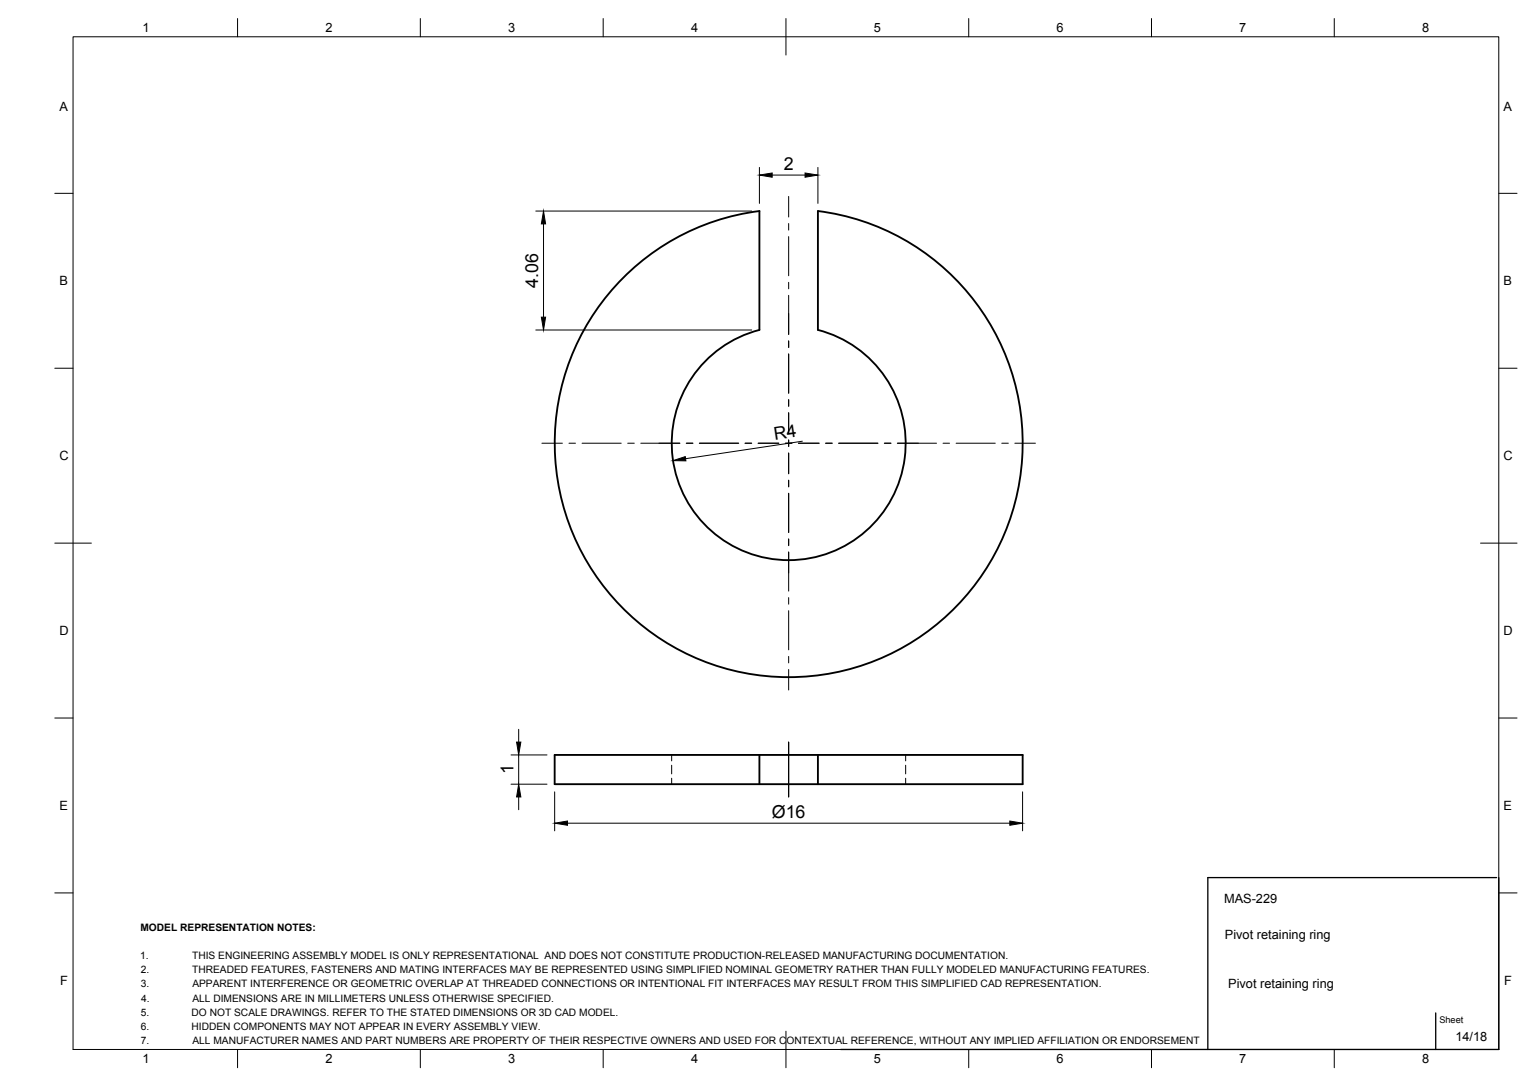
ISO-10303-21;
HEADER;
/* Generated by software containing ST-Developer
 * from STEP Tools, Inc. (www.steptools.com) 
 */

FILE_DESCRIPTION(
/* description */ ('Independently dimensioned six-bar single-leg walking-linkage demonstr
ator. Whole-mm20 crank,60 upper rocker,80/120 ternary coupler,120 lowe
r rocker,140 knee pitch and260 toe reach; ground pivots0/0,60/0,40/60.
 Seven native revolutes close both loops. Four reused native library f
amilies, fully retained shared pins and layered real spacer stacks, bo
nded rubber toe. Benchtop reference mechanism; no complete vehicle, lo
ad, gait stability, adhesive, weld, fit or life rating.'),
/* implementation_level */ '2;1');

FILE_NAME(
/* name */ 'Pivot retaining ring.step',
/* time_stamp */ '2026-11-09T20:33:14-08:00',
/* author */ (''),
/* organization */ (''),
/* preprocessor_version */ 'ST-DEVELOPER v20.2',
/* originating_system */ 'Autodesk Translation Framework v15.17.0.0',
/* authorisation */ '');

FILE_SCHEMA (('AUTOMOTIVE_DESIGN { 1 0 10303 214 3 1 1 }'));
ENDSEC;

DATA;
#10=MECHANICAL_DESIGN_GEOMETRIC_PRESENTATION_REPRESENTATION('',(#269),#4048);
#233=SHAPE_REPRESENTATION_RELATIONSHIP('SRR','None',#4157,#251);
#251=ADVANCED_BREP_SHAPE_REPRESENTATION('',(#287),#4044);
#269=STYLED_ITEM('',(#4254),#287);
#287=MANIFOLD_SOLID_BREP('Body1',#2158);
#402=PLANE('',#2574);
#403=PLANE('',#2575);
#404=PLANE('',#2576);
#405=PLANE('',#2583);
#518=FACE_OUTER_BOUND('',#694,.T.);
#519=FACE_OUTER_BOUND('',#695,.T.);
#520=FACE_OUTER_BOUND('',#696,.T.);
#521=FACE_OUTER_BOUND('',#697,.T.);
#522=FACE_OUTER_BOUND('',#698,.T.);
#523=FACE_OUTER_BOUND('',#699,.T.);
#694=EDGE_LOOP('',(#1891,#1892,#1893,#1894));
#695=EDGE_LOOP('',(#1895,#1896,#1897,#1898));
#696=EDGE_LOOP('',(#1899,#1900,#1901,#1902));
#697=EDGE_LOOP('',(#1903,#1904,#1905,#1906));
#698=EDGE_LOOP('',(#1907,#1908,#1909,#1910));
#699=EDGE_LOOP('',(#1911,#1912,#1913,#1914));
#833=LINE('',#3875,#958);
#834=LINE('',#3877,#959);
#835=LINE('',#3879,#960);
#836=LINE('',#3880,#961);
#837=LINE('',#3884,#962);
#838=LINE('',#3886,#963);
#839=LINE('',#3888,#964);
#840=LINE('',#3889,#965);
#958=VECTOR('',#3208,10.);
#959=VECTOR('',#3209,10.);
#960=VECTOR('',#3210,10.);
#961=VECTOR('',#3211,10.);
#962=VECTOR('',#3214,10.);
#963=VECTOR('',#3215,10.);
#964=VECTOR('',#3216,10.);
#965=VECTOR('',#3217,10.);
#1068=CIRCLE('',#2577,8.);
#1069=CIRCLE('',#2578,4.);
#1070=CIRCLE('',#2580,4.);
#1071=CIRCLE('',#2582,8.);
#1222=VERTEX_POINT('',#3873);
#1223=VERTEX_POINT('',#3874);
#1224=VERTEX_POINT('',#3876);
#1225=VERTEX_POINT('',#3878);
#1226=VERTEX_POINT('',#3882);
#1227=VERTEX_POINT('',#3883);
#1228=VERTEX_POINT('',#3885);
#1229=VERTEX_POINT('',#3887);
#1449=EDGE_CURVE('',#1222,#1223,#833,.T.);
#1450=EDGE_CURVE('',#1224,#1222,#834,.T.);
#1451=EDGE_CURVE('',#1225,#1224,#835,.T.);
#1452=EDGE_CURVE('',#1223,#1225,#836,.T.);
#1453=EDGE_CURVE('',#1226,#1227,#837,.T.);
#1454=EDGE_CURVE('',#1228,#1226,#838,.T.);
#1455=EDGE_CURVE('',#1229,#1228,#839,.T.);
#1456=EDGE_CURVE('',#1227,#1229,#840,.T.);
#1457=EDGE_CURVE('',#1224,#1229,#1068,.T.);
#1458=EDGE_CURVE('',#1227,#1222,#1069,.T.);
#1459=EDGE_CURVE('',#1226,#1223,#1070,.T.);
#1460=EDGE_CURVE('',#1225,#1228,#1071,.T.);
#1891=ORIENTED_EDGE('',*,*,#1449,.F.);
#1892=ORIENTED_EDGE('',*,*,#1450,.F.);
#1893=ORIENTED_EDGE('',*,*,#1451,.F.);
#1894=ORIENTED_EDGE('',*,*,#1452,.F.);
#1895=ORIENTED_EDGE('',*,*,#1453,.F.);
#1896=ORIENTED_EDGE('',*,*,#1454,.F.);
#1897=ORIENTED_EDGE('',*,*,#1455,.F.);
#1898=ORIENTED_EDGE('',*,*,#1456,.F.);
#1899=ORIENTED_EDGE('',*,*,#1456,.T.);
#1900=ORIENTED_EDGE('',*,*,#1457,.F.);
#1901=ORIENTED_EDGE('',*,*,#1450,.T.);
#1902=ORIENTED_EDGE('',*,*,#1458,.F.);
#1903=ORIENTED_EDGE('',*,*,#1453,.T.);
#1904=ORIENTED_EDGE('',*,*,#1458,.T.);
#1905=ORIENTED_EDGE('',*,*,#1449,.T.);
#1906=ORIENTED_EDGE('',*,*,#1459,.F.);
#1907=ORIENTED_EDGE('',*,*,#1455,.T.);
#1908=ORIENTED_EDGE('',*,*,#1460,.F.);
#1909=ORIENTED_EDGE('',*,*,#1451,.T.);
#1910=ORIENTED_EDGE('',*,*,#1457,.T.);
#1911=ORIENTED_EDGE('',*,*,#1454,.T.);
#1912=ORIENTED_EDGE('',*,*,#1459,.T.);
#1913=ORIENTED_EDGE('',*,*,#1452,.T.);
#1914=ORIENTED_EDGE('',*,*,#1460,.T.);
#2008=CYLINDRICAL_SURFACE('',#2579,4.);
#2009=CYLINDRICAL_SURFACE('',#2581,8.);
#2121=ADVANCED_FACE('',(#518),#402,.F.);
#2122=ADVANCED_FACE('',(#519),#403,.F.);
#2123=ADVANCED_FACE('',(#520),#404,.F.);
#2124=ADVANCED_FACE('',(#521),#2008,.F.);
#2125=ADVANCED_FACE('',(#522),#2009,.T.);
#2126=ADVANCED_FACE('',(#523),#405,.T.);
#2158=CLOSED_SHELL('',(#2121,#2122,#2123,#2124,#2125,#2126));
#2573=AXIS2_PLACEMENT_3D('',#3871,#3204,#3205);
#2574=AXIS2_PLACEMENT_3D('',#3872,#3206,#3207);
#2575=AXIS2_PLACEMENT_3D('',#3881,#3212,#3213);
#2576=AXIS2_PLACEMENT_3D('',#3890,#3218,#3219);
#2577=AXIS2_PLACEMENT_3D('',#3891,#3220,#3221);
#2578=AXIS2_PLACEMENT_3D('',#3892,#3222,#3223);
#2579=AXIS2_PLACEMENT_3D('',#3893,#3224,#3225);
#2580=AXIS2_PLACEMENT_3D('',#3894,#3226,#3227);
#2581=AXIS2_PLACEMENT_3D('',#3895,#3228,#3229);
#2582=AXIS2_PLACEMENT_3D('',#3896,#3230,#3231);
#2583=AXIS2_PLACEMENT_3D('',#3897,#3232,#3233);
#3204=DIRECTION('axis',(0.,0.,1.));
#3205=DIRECTION('refdir',(1.,0.,0.));
#3206=DIRECTION('center_axis',(-1.,0.,0.));
#3207=DIRECTION('ref_axis',(0.,1.,0.));
#3208=DIRECTION('',(0.,0.,1.));
#3209=DIRECTION('',(0.,-1.,0.));
#3210=DIRECTION('',(0.,0.,-1.));
#3211=DIRECTION('',(0.,1.,0.));
#3212=DIRECTION('center_axis',(1.,0.,0.));
#3213=DIRECTION('ref_axis',(0.,-1.,0.));
#3214=DIRECTION('',(0.,0.,-1.));
#3215=DIRECTION('',(0.,-1.,0.));
#3216=DIRECTION('',(0.,0.,1.));
#3217=DIRECTION('',(0.,1.,0.));
#3218=DIRECTION('center_axis',(0.,0.,1.));
#3219=DIRECTION('ref_axis',(1.,0.,0.));
#3220=DIRECTION('center_axis',(0.,0.,1.));
#3221=DIRECTION('ref_axis',(1.,0.,0.));
#3222=DIRECTION('center_axis',(0.,0.,-1.));
#3223=DIRECTION('ref_axis',(1.,0.,0.));
#3224=DIRECTION('center_axis',(0.,0.,1.));
#3225=DIRECTION('ref_axis',(6.12323399573677E-17,-1.,0.));
#3226=DIRECTION('center_axis',(0.,0.,-1.));
#3227=DIRECTION('ref_axis',(1.,0.,0.));
#3228=DIRECTION('center_axis',(0.,0.,1.));
#3229=DIRECTION('ref_axis',(6.12323399573677E-17,-1.,0.));
#3230=DIRECTION('center_axis',(0.,0.,1.));
#3231=DIRECTION('ref_axis',(1.,0.,0.));
#3232=DIRECTION('center_axis',(0.,0.,1.));
#3233=DIRECTION('ref_axis',(1.,0.,0.));
#3871=CARTESIAN_POINT('',(0.,0.,0.));
#3872=CARTESIAN_POINT('Origin',(-1.,0.,1.));
#3873=CARTESIAN_POINT('',(-1.,3.87298334620742,0.));
#3874=CARTESIAN_POINT('',(-1.,3.87298334620742,1.));
#3875=CARTESIAN_POINT('',(-1.,3.87298334620742,0.));
#3876=CARTESIAN_POINT('',(-1.,7.93725393319377,0.));
#3877=CARTESIAN_POINT('',(-1.,0.,0.));
#3878=CARTESIAN_POINT('',(-1.,7.93725393319377,1.));
#3879=CARTESIAN_POINT('',(-1.,7.93725393319377,0.));
#3880=CARTESIAN_POINT('',(-1.,0.,1.));
#3881=CARTESIAN_POINT('Origin',(1.,16.,1.));
#3882=CARTESIAN_POINT('',(1.,3.87298334620742,1.));
#3883=CARTESIAN_POINT('',(1.,3.87298334620742,0.));
#3884=CARTESIAN_POINT('',(1.,3.87298334620742,0.));
#3885=CARTESIAN_POINT('',(1.,7.93725393319377,1.));
#3886=CARTESIAN_POINT('',(1.,8.,1.));
#3887=CARTESIAN_POINT('',(1.,7.93725393319377,0.));
#3888=CARTESIAN_POINT('',(1.,7.93725393319377,0.));
#3889=CARTESIAN_POINT('',(1.,8.,0.));
#3890=CARTESIAN_POINT('Origin',(0.,0.,0.));
#3891=CARTESIAN_POINT('Origin',(0.,0.,0.));
#3892=CARTESIAN_POINT('Origin',(0.,0.,0.));
#3893=CARTESIAN_POINT('Origin',(0.,0.,0.));
#3894=CARTESIAN_POINT('Origin',(0.,0.,1.));
#3895=CARTESIAN_POINT('Origin',(0.,0.,0.));
#3896=CARTESIAN_POINT('Origin',(0.,0.,1.));
#3897=CARTESIAN_POINT('Origin',(0.,0.,1.));
#4024=UNCERTAINTY_MEASURE_WITH_UNIT(LENGTH_MEASURE(0.01),#4049,
'DISTANCE_ACCURACY_VALUE',
'Maximum model space distance between geometric entities at asserted c
onnectivities');
#4028=UNCERTAINTY_MEASURE_WITH_UNIT(LENGTH_MEASURE(0.01),#4049,
'DISTANCE_ACCURACY_VALUE',
'Maximum model space distance between geometric entities at asserted c
onnectivities');
#4044=(
GEOMETRIC_REPRESENTATION_CONTEXT(3)
GLOBAL_UNCERTAINTY_ASSIGNED_CONTEXT((#4024))
GLOBAL_UNIT_ASSIGNED_CONTEXT((#4049,#4051,#4052))
REPRESENTATION_CONTEXT('','3D')
);
#4048=(
GEOMETRIC_REPRESENTATION_CONTEXT(3)
GLOBAL_UNCERTAINTY_ASSIGNED_CONTEXT((#4028))
GLOBAL_UNIT_ASSIGNED_CONTEXT((#4049,#4051,#4052))
REPRESENTATION_CONTEXT('','3D')
);
#4049=(
LENGTH_UNIT()
NAMED_UNIT(*)
SI_UNIT(.MILLI.,.METRE.)
);
#4051=(
NAMED_UNIT(*)
PLANE_ANGLE_UNIT()
SI_UNIT($,.RADIAN.)
);
#4052=(
NAMED_UNIT(*)
SI_UNIT($,.STERADIAN.)
SOLID_ANGLE_UNIT()
);
#4068=SHAPE_DEFINITION_REPRESENTATION(#4087,#4157);
#4087=PRODUCT_DEFINITION_SHAPE('',$,#4177);
#4157=SHAPE_REPRESENTATION('',(#2573),#4044);
#4161=PRODUCT_DEFINITION_CONTEXT('part definition',#4220,'design');
#4177=PRODUCT_DEFINITION('Pivot retaining ring','Pivot retaining ring',
#4196,#4161);
#4196=PRODUCT_DEFINITION_FORMATION('',$,#4237);
#4220=APPLICATION_CONTEXT(
'Core Data for Automotive Mechanical Design Process');
#4221=PRODUCT_CONTEXT('part definition',#4220,'mechanical');
#4237=PRODUCT('Pivot retaining ring','Pivot retaining ring',$,(#4221));
#4254=PRESENTATION_STYLE_ASSIGNMENT((#4268));
#4268=SURFACE_STYLE_USAGE(.BOTH.,#4282);
#4282=SURFACE_SIDE_STYLE('',(#4296));
#4296=SURFACE_STYLE_FILL_AREA(#4310);
#4310=FILL_AREA_STYLE('Dark gray',(#4324));
#4324=FILL_AREA_STYLE_COLOUR('Dark gray',#4338);
#4338=COLOUR_RGB('Dark gray',0.250980392156863,0.282352941176471,0.32156862745098);
ENDSEC;
END-ISO-10303-21;
